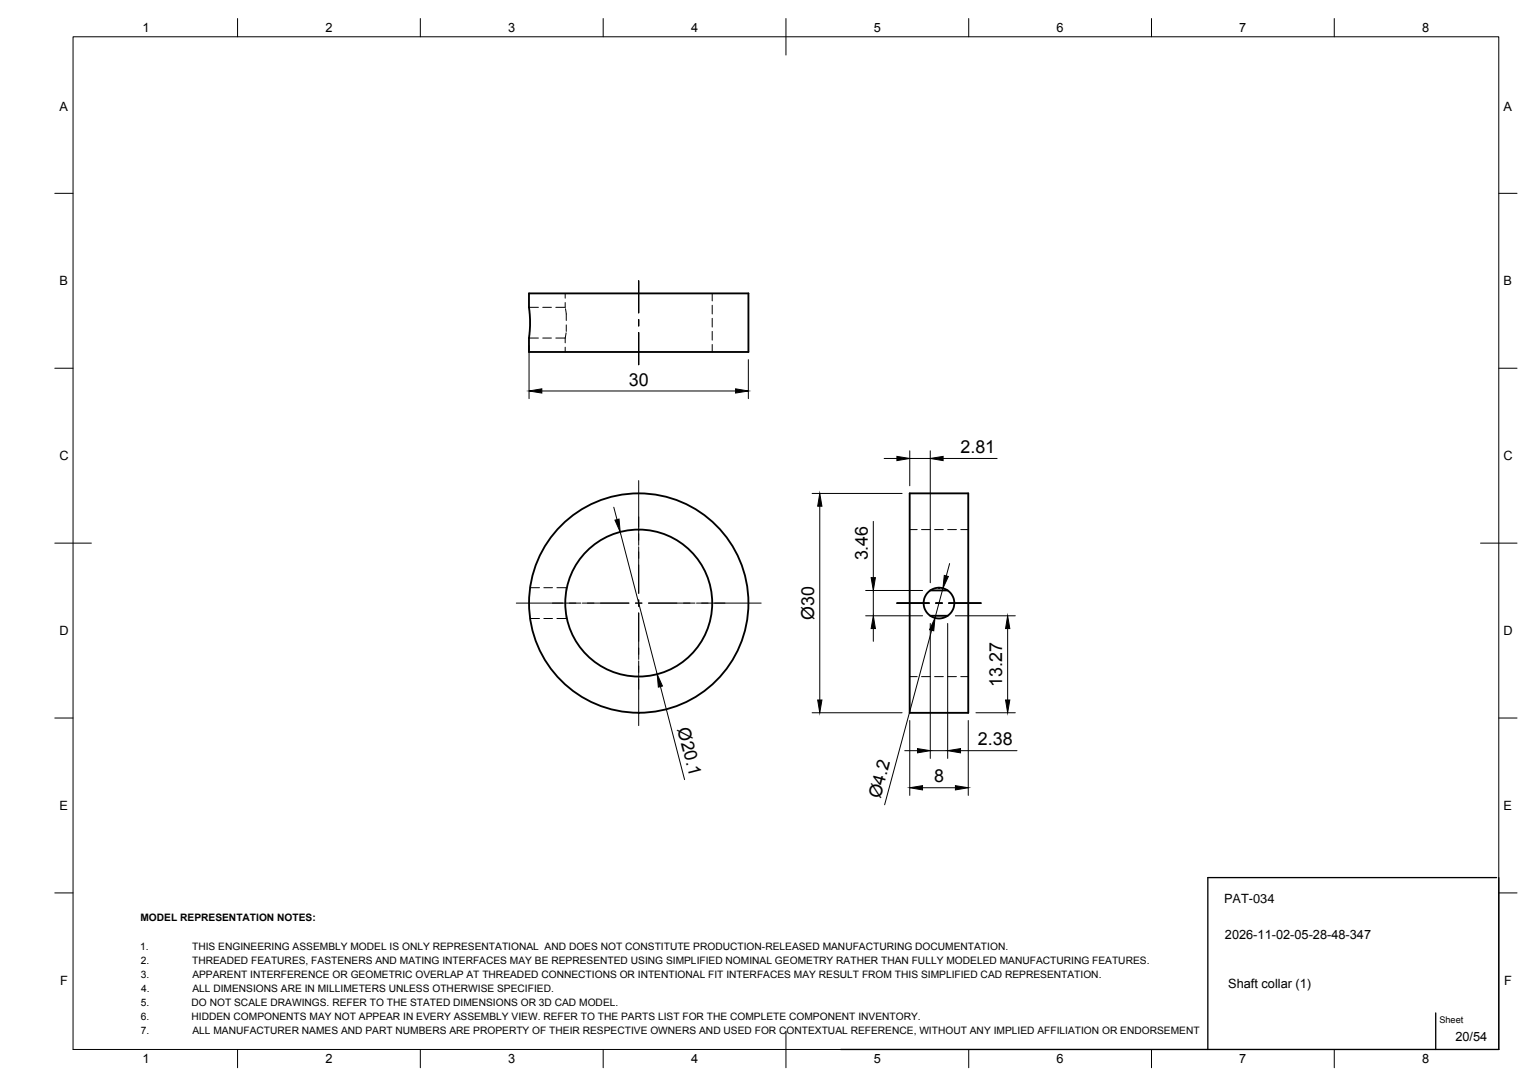
ISO-10303-21;
HEADER;
/* Generated by software containing ST-Developer
 * from STEP Tools, Inc. (www.steptools.com) 
 */

FILE_DESCRIPTION(
/* description */ ('Fatigue rig crank-slider'),
/* implementation_level */ '2;1');

FILE_NAME(
/* name */ 'Shaft collar (1).step',
/* time_stamp */ '2026-10-28T03:24:50-07:00',
/* author */ (''),
/* organization */ (''),
/* preprocessor_version */ 'ST-DEVELOPER v20.2',
/* originating_system */ 'Autodesk Translation Framework v15.17.0.0',
/* authorisation */ '');

FILE_SCHEMA (('AUTOMOTIVE_DESIGN { 1 0 10303 214 3 1 1 }'));
ENDSEC;

DATA;
#10=MECHANICAL_DESIGN_GEOMETRIC_PRESENTATION_REPRESENTATION('',(#606),#16911);
#443=B_SPLINE_CURVE_WITH_KNOTS('',3,(#14919,#14920,#14921,#14922,#14923,
#14924,#14925,#14926,#14927,#14928,#14929,#14930,#14931,#14932),
 .UNSPECIFIED.,.F.,.F.,(4,2,2,2,2,2,4),(0.756005737987028,0.793568827564648,
0.872922520054202,0.952276212543757,1.03162990503331,1.11098359752287,1.14854668710049),
 .UNSPECIFIED.);
#444=B_SPLINE_CURVE_WITH_KNOTS('',3,(#14938,#14939,#14940,#14941,#14942,
#14943,#14944,#14945,#14946,#14947,#14948,#14949,#14950,#14951,#14952,#14953,
#14954,#14955),.UNSPECIFIED.,.F.,.F.,(4,2,2,2,2,2,2,2,4),(0.,0.0792165807733633,
0.158433161546727,0.237648697074571,0.316864232602415,0.396079768130259,
0.475295303658103,0.554511884431466,0.63372846520483),.UNSPECIFIED.);
#445=B_SPLINE_CURVE_WITH_KNOTS('',3,(#14956,#14957,#14958,#14959,#14960,
#14961,#14962,#14963,#14964,#14965,#14966,#14967,#14968,#14969,#14970,#14971,
#14972,#14973),.UNSPECIFIED.,.F.,.F.,(4,2,2,2,2,2,2,2,4),(0.63372846520483,
0.712945045978193,0.792161626751556,0.8713771622794,0.950592697807245,1.02980823333509,
1.10902376886293,1.1882403496363,1.26745693040966),.UNSPECIFIED.);
#446=B_SPLINE_CURVE_WITH_KNOTS('',3,(#14976,#14977,#14978,#14979,#14980,
#14981,#14982,#14983,#14984,#14985,#14986,#14987,#14988,#14989),
 .UNSPECIFIED.,.F.,.F.,(4,2,2,2,2,2,4),(0.121154929624524,0.158718019202143,
0.238071711691698,0.317425404181252,0.396779096670807,0.476132789160362,
0.513695878737981),.UNSPECIFIED.);
#505=SHAPE_REPRESENTATION_RELATIONSHIP('SRR','None',#17146,#555);
#555=ADVANCED_BREP_SHAPE_REPRESENTATION('',(#663),#16875);
#606=STYLED_ITEM('',(#17487),#663);
#663=MANIFOLD_SOLID_BREP('Body1',#8899);
#825=FACE_BOUND('',#2103,.T.);
#826=FACE_BOUND('',#2105,.T.);
#827=FACE_BOUND('',#2107,.T.);
#828=FACE_BOUND('',#2109,.T.);
#1037=PLANE('',#9928);
#1038=PLANE('',#9933);
#1039=PLANE('',#9940);
#1040=PLANE('',#9941);
#1451=FACE_OUTER_BOUND('',#2099,.T.);
#1452=FACE_OUTER_BOUND('',#2100,.T.);
#1453=FACE_OUTER_BOUND('',#2101,.T.);
#1454=FACE_OUTER_BOUND('',#2102,.T.);
#1455=FACE_OUTER_BOUND('',#2104,.T.);
#1456=FACE_OUTER_BOUND('',#2106,.T.);
#1457=FACE_OUTER_BOUND('',#2108,.T.);
#2099=EDGE_LOOP('',(#6982,#6983));
#2100=EDGE_LOOP('',(#6984,#6985,#6986,#6987,#6988,#6989,#6990,#6991,#6992));
#2101=EDGE_LOOP('',(#6993,#6994,#6995));
#2102=EDGE_LOOP('',(#6996,#6997,#6998,#6999));
#2103=EDGE_LOOP('',(#7000,#7001,#7002,#7003));
#2104=EDGE_LOOP('',(#7004,#7005,#7006,#7007));
#2105=EDGE_LOOP('',(#7008,#7009));
#2106=EDGE_LOOP('',(#7010));
#2107=EDGE_LOOP('',(#7011));
#2108=EDGE_LOOP('',(#7012));
#2109=EDGE_LOOP('',(#7013));
#2749=LINE('',#14915,#3395);
#2750=LINE('',#14936,#3396);
#2751=LINE('',#14991,#3397);
#2752=LINE('',#14996,#3398);
#2753=LINE('',#15002,#3399);
#3395=VECTOR('',#11727,1.);
#3396=VECTOR('',#11734,0.21);
#3397=VECTOR('',#11739,1.);
#3398=VECTOR('',#11744,1.005);
#3399=VECTOR('',#11751,1.5);
#3928=CIRCLE('',#9929,0.21);
#3929=CIRCLE('',#9931,0.21);
#3930=CIRCLE('',#9932,0.21);
#3931=CIRCLE('',#9935,1.005);
#3932=CIRCLE('',#9936,1.005);
#3933=CIRCLE('',#9938,1.5);
#3934=CIRCLE('',#9939,1.5);
#4486=VERTEX_POINT('',#14913);
#4487=VERTEX_POINT('',#14914);
#4488=VERTEX_POINT('',#14918);
#4489=VERTEX_POINT('',#14933);
#4490=VERTEX_POINT('',#14935);
#4491=VERTEX_POINT('',#14937);
#4492=VERTEX_POINT('',#14974);
#4493=VERTEX_POINT('',#14993);
#4494=VERTEX_POINT('',#14995);
#4495=VERTEX_POINT('',#14999);
#4496=VERTEX_POINT('',#15001);
#5389=EDGE_CURVE('',#4486,#4487,#2749,.T.);
#5390=EDGE_CURVE('',#4486,#4487,#3928,.T.);
#5391=EDGE_CURVE('',#4488,#4486,#443,.T.);
#5392=EDGE_CURVE('',#4489,#4488,#3929,.T.);
#5393=EDGE_CURVE('',#4489,#4490,#2750,.T.);
#5394=EDGE_CURVE('',#4491,#4490,#444,.T.);
#5395=EDGE_CURVE('',#4490,#4491,#445,.T.);
#5396=EDGE_CURVE('',#4492,#4489,#3930,.T.);
#5397=EDGE_CURVE('',#4487,#4492,#446,.T.);
#5398=EDGE_CURVE('',#4492,#4488,#2751,.T.);
#5399=EDGE_CURVE('',#4493,#4493,#3931,.T.);
#5400=EDGE_CURVE('',#4493,#4494,#2752,.T.);
#5401=EDGE_CURVE('',#4494,#4494,#3932,.T.);
#5402=EDGE_CURVE('',#4495,#4495,#3933,.T.);
#5403=EDGE_CURVE('',#4495,#4496,#2753,.T.);
#5404=EDGE_CURVE('',#4496,#4496,#3934,.T.);
#6982=ORIENTED_EDGE('',*,*,#5389,.F.);
#6983=ORIENTED_EDGE('',*,*,#5390,.T.);
#6984=ORIENTED_EDGE('',*,*,#5391,.F.);
#6985=ORIENTED_EDGE('',*,*,#5392,.F.);
#6986=ORIENTED_EDGE('',*,*,#5393,.T.);
#6987=ORIENTED_EDGE('',*,*,#5394,.F.);
#6988=ORIENTED_EDGE('',*,*,#5395,.F.);
#6989=ORIENTED_EDGE('',*,*,#5393,.F.);
#6990=ORIENTED_EDGE('',*,*,#5396,.F.);
#6991=ORIENTED_EDGE('',*,*,#5397,.F.);
#6992=ORIENTED_EDGE('',*,*,#5390,.F.);
#6993=ORIENTED_EDGE('',*,*,#5398,.F.);
#6994=ORIENTED_EDGE('',*,*,#5396,.T.);
#6995=ORIENTED_EDGE('',*,*,#5392,.T.);
#6996=ORIENTED_EDGE('',*,*,#5399,.F.);
#6997=ORIENTED_EDGE('',*,*,#5400,.T.);
#6998=ORIENTED_EDGE('',*,*,#5401,.T.);
#6999=ORIENTED_EDGE('',*,*,#5400,.F.);
#7000=ORIENTED_EDGE('',*,*,#5397,.T.);
#7001=ORIENTED_EDGE('',*,*,#5398,.T.);
#7002=ORIENTED_EDGE('',*,*,#5391,.T.);
#7003=ORIENTED_EDGE('',*,*,#5389,.T.);
#7004=ORIENTED_EDGE('',*,*,#5402,.F.);
#7005=ORIENTED_EDGE('',*,*,#5403,.T.);
#7006=ORIENTED_EDGE('',*,*,#5404,.T.);
#7007=ORIENTED_EDGE('',*,*,#5403,.F.);
#7008=ORIENTED_EDGE('',*,*,#5394,.T.);
#7009=ORIENTED_EDGE('',*,*,#5395,.T.);
#7010=ORIENTED_EDGE('',*,*,#5402,.T.);
#7011=ORIENTED_EDGE('',*,*,#5399,.T.);
#7012=ORIENTED_EDGE('',*,*,#5404,.F.);
#7013=ORIENTED_EDGE('',*,*,#5401,.F.);
#8281=CYLINDRICAL_SURFACE('',#9930,0.21);
#8282=CYLINDRICAL_SURFACE('',#9934,1.005);
#8283=CYLINDRICAL_SURFACE('',#9937,1.5);
#8589=ADVANCED_FACE('',(#1451),#1037,.T.);
#8590=ADVANCED_FACE('',(#1452),#8281,.F.);
#8591=ADVANCED_FACE('',(#1453),#1038,.T.);
#8592=ADVANCED_FACE('',(#1454,#825),#8282,.F.);
#8593=ADVANCED_FACE('',(#1455,#826),#8283,.T.);
#8594=ADVANCED_FACE('',(#1456,#827),#1039,.T.);
#8595=ADVANCED_FACE('',(#1457,#828),#1040,.F.);
#8899=CLOSED_SHELL('',(#8589,#8590,#8591,#8592,#8593,#8594,#8595));
#9927=AXIS2_PLACEMENT_3D('',#14911,#11723,#11724);
#9928=AXIS2_PLACEMENT_3D('',#14912,#11725,#11726);
#9929=AXIS2_PLACEMENT_3D('',#14916,#11728,#11729);
#9930=AXIS2_PLACEMENT_3D('',#14917,#11730,#11731);
#9931=AXIS2_PLACEMENT_3D('',#14934,#11732,#11733);
#9932=AXIS2_PLACEMENT_3D('',#14975,#11735,#11736);
#9933=AXIS2_PLACEMENT_3D('',#14990,#11737,#11738);
#9934=AXIS2_PLACEMENT_3D('',#14992,#11740,#11741);
#9935=AXIS2_PLACEMENT_3D('',#14994,#11742,#11743);
#9936=AXIS2_PLACEMENT_3D('',#14997,#11745,#11746);
#9937=AXIS2_PLACEMENT_3D('',#14998,#11747,#11748);
#9938=AXIS2_PLACEMENT_3D('',#15000,#11749,#11750);
#9939=AXIS2_PLACEMENT_3D('',#15003,#11752,#11753);
#9940=AXIS2_PLACEMENT_3D('',#15004,#11754,#11755);
#9941=AXIS2_PLACEMENT_3D('',#15005,#11756,#11757);
#11723=DIRECTION('axis',(0.,0.,1.));
#11724=DIRECTION('refdir',(1.,0.,0.));
#11725=DIRECTION('center_axis',(0.,0.,1.));
#11726=DIRECTION('ref_axis',(1.,0.,0.));
#11727=DIRECTION('',(0.,1.,0.));
#11728=DIRECTION('center_axis',(0.,0.,1.));
#11729=DIRECTION('ref_axis',(1.,0.,0.));
#11730=DIRECTION('center_axis',(0.,0.,1.));
#11731=DIRECTION('ref_axis',(1.,0.,0.));
#11732=DIRECTION('center_axis',(0.,0.,1.));
#11733=DIRECTION('ref_axis',(1.,0.,0.));
#11734=DIRECTION('',(0.,0.,1.));
#11735=DIRECTION('center_axis',(0.,0.,1.));
#11736=DIRECTION('ref_axis',(1.,0.,0.));
#11737=DIRECTION('center_axis',(0.,0.,1.));
#11738=DIRECTION('ref_axis',(1.,0.,0.));
#11739=DIRECTION('',(0.,-1.,0.));
#11740=DIRECTION('center_axis',(0.,1.,0.));
#11741=DIRECTION('ref_axis',(1.,0.,0.));
#11742=DIRECTION('center_axis',(0.,-1.,0.));
#11743=DIRECTION('ref_axis',(1.,0.,0.));
#11744=DIRECTION('',(0.,-1.,0.));
#11745=DIRECTION('center_axis',(0.,-1.,0.));
#11746=DIRECTION('ref_axis',(1.,0.,0.));
#11747=DIRECTION('center_axis',(0.,1.,0.));
#11748=DIRECTION('ref_axis',(1.,0.,0.));
#11749=DIRECTION('center_axis',(0.,1.,0.));
#11750=DIRECTION('ref_axis',(1.,0.,0.));
#11751=DIRECTION('',(0.,-1.,0.));
#11752=DIRECTION('center_axis',(0.,1.,0.));
#11753=DIRECTION('ref_axis',(1.,0.,0.));
#11754=DIRECTION('center_axis',(0.,1.,0.));
#11755=DIRECTION('ref_axis',(1.,0.,0.));
#11756=DIRECTION('center_axis',(0.,1.,0.));
#11757=DIRECTION('ref_axis',(1.,0.,0.));
#14911=CARTESIAN_POINT('',(0.,0.,0.));
#14912=CARTESIAN_POINT('Origin',(0.,-4.15,12.99));
#14913=CARTESIAN_POINT('',(0.172988438920051,-4.26905880899792,12.99));
#14914=CARTESIAN_POINT('',(0.172988438920051,-4.03094119100208,12.99));
#14915=CARTESIAN_POINT('',(0.172988438920051,-4.55,12.99));
#14916=CARTESIAN_POINT('Origin',(0.,-4.15,12.99));
#14917=CARTESIAN_POINT('Origin',(0.,-4.15,12.99));
#14918=CARTESIAN_POINT('',(-0.172988438920051,-4.26905880899792,12.99));
#14919=CARTESIAN_POINT('Ctrl Pts',(-0.172988438920051,-4.26905880899792,
12.99));
#14920=CARTESIAN_POINT('Ctrl Pts',(-0.16559486531131,-4.2798014223953,12.9912919219764));
#14921=CARTESIAN_POINT('Ctrl Pts',(-0.157297138725605,-4.28968770937275,
12.9926539494391));
#14922=CARTESIAN_POINT('Ctrl Pts',(-0.129892073845076,-4.31709277425327,
12.9967480843909));
#14923=CARTESIAN_POINT('Ctrl Pts',(-0.106330167759284,-4.33324205633295,
12.9996958932764));
#14924=CARTESIAN_POINT('Ctrl Pts',(-0.05461290463241,-4.35469779396491,
13.0038502947236));
#14925=CARTESIAN_POINT('Ctrl Pts',(-0.0264512308298516,-4.36,13.005));
#14926=CARTESIAN_POINT('Ctrl Pts',(0.0264512308298515,-4.36,13.005));
#14927=CARTESIAN_POINT('Ctrl Pts',(0.0546129046324099,-4.35469779396491,
13.0038502947236));
#14928=CARTESIAN_POINT('Ctrl Pts',(0.106330167759284,-4.33324205633295,
12.9996958932764));
#14929=CARTESIAN_POINT('Ctrl Pts',(0.129892073845076,-4.31709277425327,
12.9967480843909));
#14930=CARTESIAN_POINT('Ctrl Pts',(0.157297138725605,-4.28968770937275,
12.992653949439));
#14931=CARTESIAN_POINT('Ctrl Pts',(0.165594865311311,-4.2798014223953,12.9912919219764));
#14932=CARTESIAN_POINT('Ctrl Pts',(0.172988438920051,-4.26905880899792,
12.99));
#14933=CARTESIAN_POINT('',(-0.21,-4.15,12.99));
#14934=CARTESIAN_POINT('Origin',(0.,-4.15,12.99));
#14935=CARTESIAN_POINT('',(-0.21,-4.15,13.4852272553384));
#14936=CARTESIAN_POINT('',(-0.21,-4.15,12.99));
#14937=CARTESIAN_POINT('',(0.21,-4.15,13.4852272553384));
#14938=CARTESIAN_POINT('Ctrl Pts',(0.21,-4.15,13.4852272553384));
#14939=CARTESIAN_POINT('Ctrl Pts',(0.21,-4.17640552692446,13.4852272553384));
#14940=CARTESIAN_POINT('Ctrl Pts',(0.204715737269596,-4.20454707409071,
13.4860041595441));
#14941=CARTESIAN_POINT('Ctrl Pts',(0.183273763036332,-4.25627626890513,
13.4888007328232));
#14942=CARTESIAN_POINT('Ctrl Pts',(0.167117923970394,-4.27986692412796,
13.4907789715758));
#14943=CARTESIAN_POINT('Ctrl Pts',(0.129867169887369,-4.31711767821098,
13.4944848114133));
#14944=CARTESIAN_POINT('Ctrl Pts',(0.106276408305765,-4.33327371000135,
13.4964545565713));
#14945=CARTESIAN_POINT('Ctrl Pts',(0.0545468514059003,-4.35471582482622,
13.4992316551565));
#14946=CARTESIAN_POINT('Ctrl Pts',(0.0264051785092814,-4.36,13.5));
#14947=CARTESIAN_POINT('Ctrl Pts',(-0.0264051785092814,-4.36,13.5));
#14948=CARTESIAN_POINT('Ctrl Pts',(-0.0545468514059002,-4.35471582482622,
13.4992316551565));
#14949=CARTESIAN_POINT('Ctrl Pts',(-0.106276408305765,-4.33327371000135,
13.4964545565713));
#14950=CARTESIAN_POINT('Ctrl Pts',(-0.129867169887369,-4.31711767821098,
13.4944848114133));
#14951=CARTESIAN_POINT('Ctrl Pts',(-0.167117923970394,-4.27986692412796,
13.4907789715758));
#14952=CARTESIAN_POINT('Ctrl Pts',(-0.183273763036332,-4.25627626890513,
13.4888007328232));
#14953=CARTESIAN_POINT('Ctrl Pts',(-0.204715737269596,-4.20454707409071,
13.4860041595441));
#14954=CARTESIAN_POINT('Ctrl Pts',(-0.21,-4.17640552692446,13.4852272553384));
#14955=CARTESIAN_POINT('Ctrl Pts',(-0.21,-4.15,13.4852272553384));
#14956=CARTESIAN_POINT('Ctrl Pts',(-0.21,-4.15,13.4852272553384));
#14957=CARTESIAN_POINT('Ctrl Pts',(-0.21,-4.12359447307555,13.4852272553384));
#14958=CARTESIAN_POINT('Ctrl Pts',(-0.204715737269596,-4.09545292590929,
13.4860041595441));
#14959=CARTESIAN_POINT('Ctrl Pts',(-0.183273763036332,-4.04372373109487,
13.4888007328232));
#14960=CARTESIAN_POINT('Ctrl Pts',(-0.167117923970394,-4.02013307587204,
13.4907789715758));
#14961=CARTESIAN_POINT('Ctrl Pts',(-0.129867169887369,-3.98288232178902,
13.4944848114133));
#14962=CARTESIAN_POINT('Ctrl Pts',(-0.106276408305765,-3.96672628999865,
13.4964545565713));
#14963=CARTESIAN_POINT('Ctrl Pts',(-0.0545468514059,-3.94528417517378,13.4992316551565));
#14964=CARTESIAN_POINT('Ctrl Pts',(-0.0264051785092814,-3.94,13.5));
#14965=CARTESIAN_POINT('Ctrl Pts',(0.0264051785092813,-3.94,13.5));
#14966=CARTESIAN_POINT('Ctrl Pts',(0.0545468514058999,-3.94528417517378,
13.4992316551565));
#14967=CARTESIAN_POINT('Ctrl Pts',(0.106276408305765,-3.96672628999865,
13.4964545565713));
#14968=CARTESIAN_POINT('Ctrl Pts',(0.129867169887369,-3.98288232178902,
13.4944848114133));
#14969=CARTESIAN_POINT('Ctrl Pts',(0.167117923970394,-4.02013307587204,
13.4907789715758));
#14970=CARTESIAN_POINT('Ctrl Pts',(0.183273763036331,-4.04372373109487,
13.4888007328232));
#14971=CARTESIAN_POINT('Ctrl Pts',(0.204715737269596,-4.09545292590929,
13.4860041595441));
#14972=CARTESIAN_POINT('Ctrl Pts',(0.21,-4.12359447307555,13.4852272553384));
#14973=CARTESIAN_POINT('Ctrl Pts',(0.21,-4.15,13.4852272553384));
#14974=CARTESIAN_POINT('',(-0.172988438920051,-4.03094119100208,12.99));
#14975=CARTESIAN_POINT('Origin',(0.,-4.15,12.99));
#14976=CARTESIAN_POINT('Ctrl Pts',(0.172988438920051,-4.03094119100208,
12.99));
#14977=CARTESIAN_POINT('Ctrl Pts',(0.165594865311311,-4.0201985776047,12.9912919219764));
#14978=CARTESIAN_POINT('Ctrl Pts',(0.157297138725604,-4.01031229062725,
12.9926539494391));
#14979=CARTESIAN_POINT('Ctrl Pts',(0.129892073845076,-3.98290722574673,
12.9967480843909));
#14980=CARTESIAN_POINT('Ctrl Pts',(0.106330167759284,-3.96675794366705,
12.9996958932764));
#14981=CARTESIAN_POINT('Ctrl Pts',(0.0546129046324106,-3.94530220603509,
13.0038502947236));
#14982=CARTESIAN_POINT('Ctrl Pts',(0.0264512308298516,-3.94,13.005));
#14983=CARTESIAN_POINT('Ctrl Pts',(-0.0264512308298516,-3.94,13.005));
#14984=CARTESIAN_POINT('Ctrl Pts',(-0.0546129046324106,-3.94530220603509,
13.0038502947236));
#14985=CARTESIAN_POINT('Ctrl Pts',(-0.106330167759284,-3.96675794366705,
12.9996958932764));
#14986=CARTESIAN_POINT('Ctrl Pts',(-0.129892073845076,-3.98290722574673,
12.9967480843909));
#14987=CARTESIAN_POINT('Ctrl Pts',(-0.157297138725604,-4.01031229062725,
12.992653949439));
#14988=CARTESIAN_POINT('Ctrl Pts',(-0.165594865311311,-4.0201985776047,
12.9912919219764));
#14989=CARTESIAN_POINT('Ctrl Pts',(-0.172988438920051,-4.03094119100208,
12.99));
#14990=CARTESIAN_POINT('Origin',(0.,-4.15,12.99));
#14991=CARTESIAN_POINT('',(-0.172988438920051,-4.55,12.99));
#14992=CARTESIAN_POINT('Origin',(0.,-4.55,12.));
#14993=CARTESIAN_POINT('',(-1.005,-3.75,12.));
#14994=CARTESIAN_POINT('Origin',(0.,-3.75,12.));
#14995=CARTESIAN_POINT('',(-1.005,-4.55,12.));
#14996=CARTESIAN_POINT('',(-1.005,-4.55,12.));
#14997=CARTESIAN_POINT('Origin',(0.,-4.55,12.));
#14998=CARTESIAN_POINT('Origin',(0.,-4.55,12.));
#14999=CARTESIAN_POINT('',(-1.5,-3.75,12.));
#15000=CARTESIAN_POINT('Origin',(0.,-3.75,12.));
#15001=CARTESIAN_POINT('',(-1.5,-4.55,12.));
#15002=CARTESIAN_POINT('',(-1.5,-4.55,12.));
#15003=CARTESIAN_POINT('Origin',(0.,-4.55,12.));
#15004=CARTESIAN_POINT('Origin',(0.,-3.75,12.));
#15005=CARTESIAN_POINT('Origin',(0.,-4.55,12.));
#16816=UNCERTAINTY_MEASURE_WITH_UNIT(LENGTH_MEASURE(0.001),#16912,
'DISTANCE_ACCURACY_VALUE',
'Maximum model space distance between geometric entities at asserted c
onnectivities');
#16852=UNCERTAINTY_MEASURE_WITH_UNIT(LENGTH_MEASURE(0.001),#16912,
'DISTANCE_ACCURACY_VALUE',
'Maximum model space distance between geometric entities at asserted c
onnectivities');
#16875=(
GEOMETRIC_REPRESENTATION_CONTEXT(3)
GLOBAL_UNCERTAINTY_ASSIGNED_CONTEXT((#16816))
GLOBAL_UNIT_ASSIGNED_CONTEXT((#16912,#16914,#16915))
REPRESENTATION_CONTEXT('','3D')
);
#16911=(
GEOMETRIC_REPRESENTATION_CONTEXT(3)
GLOBAL_UNCERTAINTY_ASSIGNED_CONTEXT((#16852))
GLOBAL_UNIT_ASSIGNED_CONTEXT((#16912,#16914,#16915))
REPRESENTATION_CONTEXT('','3D')
);
#16912=(
LENGTH_UNIT()
NAMED_UNIT(*)
SI_UNIT(.CENTI.,.METRE.)
);
#16914=(
NAMED_UNIT(*)
PLANE_ANGLE_UNIT()
SI_UNIT($,.RADIAN.)
);
#16915=(
NAMED_UNIT(*)
SI_UNIT($,.STERADIAN.)
SOLID_ANGLE_UNIT()
);
#16938=SHAPE_DEFINITION_REPRESENTATION(#16998,#17146);
#16998=PRODUCT_DEFINITION_SHAPE('',$,#17205);
#17146=SHAPE_REPRESENTATION('',(#9927),#16875);
#17182=PRODUCT_DEFINITION_CONTEXT('part definition',#17358,'design');
#17205=PRODUCT_DEFINITION('Shaft collar (1)','Shaft collar (1)',#17263,#17182);
#17263=PRODUCT_DEFINITION_FORMATION('',$,#17382);
#17358=APPLICATION_CONTEXT(
'Core Data for Automotive Mechanical Design Process');
#17359=PRODUCT_CONTEXT('part definition',#17358,'mechanical');
#17382=PRODUCT('Shaft collar (1)','Shaft collar (1)','Shaft collar (1)',(#17359));
#17481=COLOUR_RGB('Grey',0.48,0.52,0.57);
#17482=FILL_AREA_STYLE_COLOUR('',#17481);
#17483=FILL_AREA_STYLE('',(#17482));
#17484=SURFACE_STYLE_FILL_AREA(#17483);
#17485=SURFACE_SIDE_STYLE('',(#17484));
#17486=SURFACE_STYLE_USAGE(.BOTH.,#17485);
#17487=PRESENTATION_STYLE_ASSIGNMENT((#17486));
ENDSEC;
END-ISO-10303-21;
